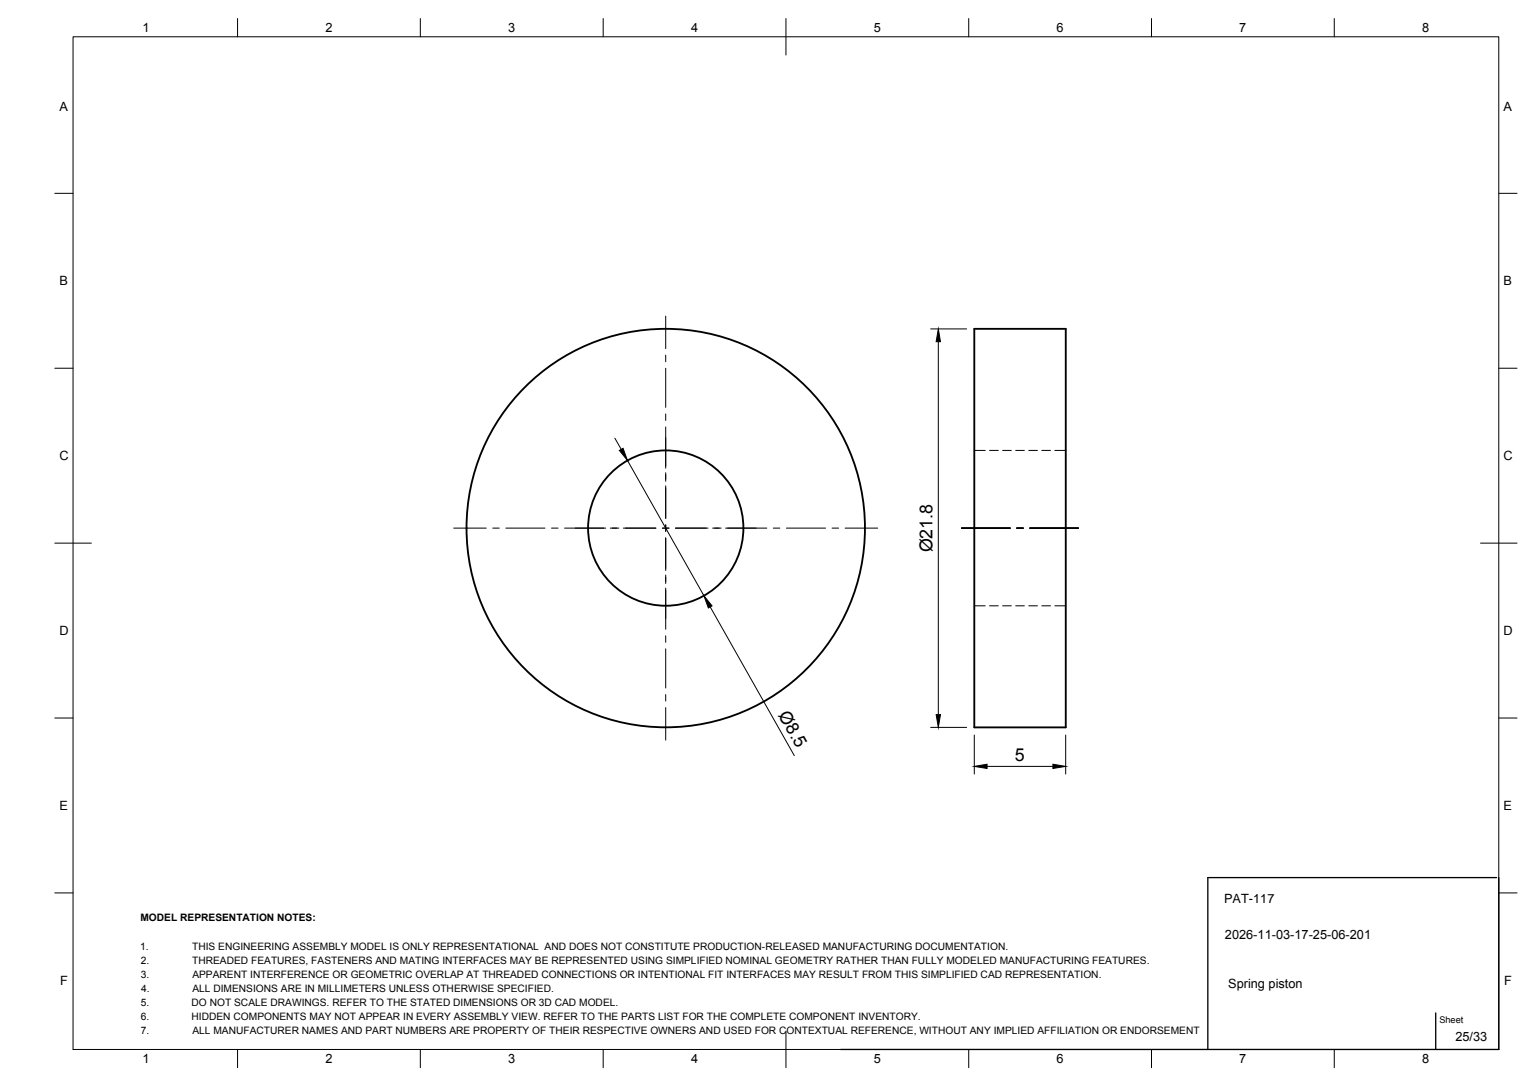
ISO-10303-21;
HEADER;
/* Generated by software containing ST-Developer
 * from STEP Tools, Inc. (www.steptools.com) 
 */

FILE_DESCRIPTION(
/* description */ ('Counterbalanced vertical column'),
/* implementation_level */ '2;1');

FILE_NAME(
/* name */ 'Spring piston.step',
/* time_stamp */ '2026-10-29T16:47:22-07:00',
/* author */ (''),
/* organization */ (''),
/* preprocessor_version */ 'ST-DEVELOPER v20.2',
/* originating_system */ 'Autodesk Translation Framework v15.17.0.0',
/* authorisation */ '');

FILE_SCHEMA (('AUTOMOTIVE_DESIGN { 1 0 10303 214 3 1 1 }'));
ENDSEC;

DATA;
#10=MECHANICAL_DESIGN_GEOMETRIC_PRESENTATION_REPRESENTATION('',(#374),#15040);
#304=SHAPE_REPRESENTATION_RELATIONSHIP('SRR','None',#15209,#339);
#339=ADVANCED_BREP_SHAPE_REPRESENTATION('',(#407),#15028);
#374=STYLED_ITEM('',(#15457),#407);
#407=MANIFOLD_SOLID_BREP('Body1',#7099);
#514=FACE_BOUND('',#1625,.T.);
#515=FACE_BOUND('',#1627,.T.);
#741=PLANE('',#7990);
#742=PLANE('',#7991);
#1119=FACE_OUTER_BOUND('',#1622,.T.);
#1120=FACE_OUTER_BOUND('',#1623,.T.);
#1121=FACE_OUTER_BOUND('',#1624,.T.);
#1122=FACE_OUTER_BOUND('',#1626,.T.);
#1622=EDGE_LOOP('',(#6090,#6091,#6092,#6093));
#1623=EDGE_LOOP('',(#6094,#6095,#6096,#6097));
#1624=EDGE_LOOP('',(#6098));
#1625=EDGE_LOOP('',(#6099));
#1626=EDGE_LOOP('',(#6100));
#1627=EDGE_LOOP('',(#6101));
#2235=LINE('',#14382,#2906);
#2236=LINE('',#14388,#2907);
#2906=VECTOR('',#9681,0.425);
#2907=VECTOR('',#9688,1.09);
#3251=CIRCLE('',#7985,0.425);
#3252=CIRCLE('',#7986,0.425);
#3253=CIRCLE('',#7988,1.09);
#3254=CIRCLE('',#7989,1.09);
#3736=VERTEX_POINT('',#14379);
#3737=VERTEX_POINT('',#14381);
#3738=VERTEX_POINT('',#14385);
#3739=VERTEX_POINT('',#14387);
#4546=EDGE_CURVE('',#3736,#3736,#3251,.T.);
#4547=EDGE_CURVE('',#3736,#3737,#2235,.T.);
#4548=EDGE_CURVE('',#3737,#3737,#3252,.T.);
#4549=EDGE_CURVE('',#3738,#3738,#3253,.T.);
#4550=EDGE_CURVE('',#3738,#3739,#2236,.T.);
#4551=EDGE_CURVE('',#3739,#3739,#3254,.T.);
#6090=ORIENTED_EDGE('',*,*,#4546,.F.);
#6091=ORIENTED_EDGE('',*,*,#4547,.T.);
#6092=ORIENTED_EDGE('',*,*,#4548,.F.);
#6093=ORIENTED_EDGE('',*,*,#4547,.F.);
#6094=ORIENTED_EDGE('',*,*,#4549,.F.);
#6095=ORIENTED_EDGE('',*,*,#4550,.T.);
#6096=ORIENTED_EDGE('',*,*,#4551,.T.);
#6097=ORIENTED_EDGE('',*,*,#4550,.F.);
#6098=ORIENTED_EDGE('',*,*,#4549,.T.);
#6099=ORIENTED_EDGE('',*,*,#4548,.T.);
#6100=ORIENTED_EDGE('',*,*,#4551,.F.);
#6101=ORIENTED_EDGE('',*,*,#4546,.T.);
#6648=CYLINDRICAL_SURFACE('',#7984,0.425);
#6649=CYLINDRICAL_SURFACE('',#7987,1.09);
#6961=ADVANCED_FACE('',(#1119),#6648,.F.);
#6962=ADVANCED_FACE('',(#1120),#6649,.T.);
#6963=ADVANCED_FACE('',(#1121,#514),#741,.T.);
#6964=ADVANCED_FACE('',(#1122,#515),#742,.F.);
#7099=CLOSED_SHELL('',(#6961,#6962,#6963,#6964));
#7983=AXIS2_PLACEMENT_3D('',#14377,#9675,#9676);
#7984=AXIS2_PLACEMENT_3D('',#14378,#9677,#9678);
#7985=AXIS2_PLACEMENT_3D('',#14380,#9679,#9680);
#7986=AXIS2_PLACEMENT_3D('',#14383,#9682,#9683);
#7987=AXIS2_PLACEMENT_3D('',#14384,#9684,#9685);
#7988=AXIS2_PLACEMENT_3D('',#14386,#9686,#9687);
#7989=AXIS2_PLACEMENT_3D('',#14389,#9689,#9690);
#7990=AXIS2_PLACEMENT_3D('',#14390,#9691,#9692);
#7991=AXIS2_PLACEMENT_3D('',#14391,#9693,#9694);
#9675=DIRECTION('axis',(0.,0.,1.));
#9676=DIRECTION('refdir',(1.,0.,0.));
#9677=DIRECTION('center_axis',(0.,0.,1.));
#9678=DIRECTION('ref_axis',(1.,0.,0.));
#9679=DIRECTION('center_axis',(0.,0.,1.));
#9680=DIRECTION('ref_axis',(1.,0.,0.));
#9681=DIRECTION('',(0.,0.,1.));
#9682=DIRECTION('center_axis',(0.,0.,-1.));
#9683=DIRECTION('ref_axis',(1.,0.,0.));
#9684=DIRECTION('center_axis',(0.,0.,1.));
#9685=DIRECTION('ref_axis',(1.,0.,0.));
#9686=DIRECTION('center_axis',(0.,0.,1.));
#9687=DIRECTION('ref_axis',(1.,0.,0.));
#9688=DIRECTION('',(0.,0.,-1.));
#9689=DIRECTION('center_axis',(0.,0.,1.));
#9690=DIRECTION('ref_axis',(1.,0.,0.));
#9691=DIRECTION('center_axis',(0.,0.,1.));
#9692=DIRECTION('ref_axis',(1.,0.,0.));
#9693=DIRECTION('center_axis',(0.,0.,1.));
#9694=DIRECTION('ref_axis',(1.,0.,0.));
#14377=CARTESIAN_POINT('',(0.,0.,0.));
#14378=CARTESIAN_POINT('Origin',(-7.,0.,4.9));
#14379=CARTESIAN_POINT('',(-7.425,-5.20474889637625E-17,5.));
#14380=CARTESIAN_POINT('Origin',(-7.,0.,5.));
#14381=CARTESIAN_POINT('',(-7.425,5.20474889637625E-17,5.5));
#14382=CARTESIAN_POINT('',(-7.425,-5.20474889637625E-17,4.9));
#14383=CARTESIAN_POINT('Origin',(-7.,0.,5.5));
#14384=CARTESIAN_POINT('Origin',(-7.,0.,5.));
#14385=CARTESIAN_POINT('',(-8.09,-1.33486501107061E-16,5.5));
#14386=CARTESIAN_POINT('Origin',(-7.,0.,5.5));
#14387=CARTESIAN_POINT('',(-8.09,-1.33486501107061E-16,5.));
#14388=CARTESIAN_POINT('',(-8.09,-1.33486501107061E-16,5.));
#14389=CARTESIAN_POINT('Origin',(-7.,0.,5.));
#14390=CARTESIAN_POINT('Origin',(-7.,0.,5.5));
#14391=CARTESIAN_POINT('Origin',(-7.,0.,5.));
#14988=UNCERTAINTY_MEASURE_WITH_UNIT(LENGTH_MEASURE(0.001),#15041,
'DISTANCE_ACCURACY_VALUE',
'Maximum model space distance between geometric entities at asserted c
onnectivities');
#15000=UNCERTAINTY_MEASURE_WITH_UNIT(LENGTH_MEASURE(0.001),#15041,
'DISTANCE_ACCURACY_VALUE',
'Maximum model space distance between geometric entities at asserted c
onnectivities');
#15028=(
GEOMETRIC_REPRESENTATION_CONTEXT(3)
GLOBAL_UNCERTAINTY_ASSIGNED_CONTEXT((#14988))
GLOBAL_UNIT_ASSIGNED_CONTEXT((#15041,#15043,#15044))
REPRESENTATION_CONTEXT('','3D')
);
#15040=(
GEOMETRIC_REPRESENTATION_CONTEXT(3)
GLOBAL_UNCERTAINTY_ASSIGNED_CONTEXT((#15000))
GLOBAL_UNIT_ASSIGNED_CONTEXT((#15041,#15043,#15044))
REPRESENTATION_CONTEXT('','3D')
);
#15041=(
LENGTH_UNIT()
NAMED_UNIT(*)
SI_UNIT(.CENTI.,.METRE.)
);
#15043=(
NAMED_UNIT(*)
PLANE_ANGLE_UNIT()
SI_UNIT($,.RADIAN.)
);
#15044=(
NAMED_UNIT(*)
SI_UNIT($,.STERADIAN.)
SOLID_ANGLE_UNIT()
);
#15072=SHAPE_DEFINITION_REPRESENTATION(#15111,#15209);
#15111=PRODUCT_DEFINITION_SHAPE('',$,#15249);
#15209=SHAPE_REPRESENTATION('',(#7983),#15028);
#15221=PRODUCT_DEFINITION_CONTEXT('part definition',#15340,'design');
#15249=PRODUCT_DEFINITION('Spring piston','Spring piston',#15288,#15221);
#15288=PRODUCT_DEFINITION_FORMATION('',$,#15369);
#15340=APPLICATION_CONTEXT(
'Core Data for Automotive Mechanical Design Process');
#15341=PRODUCT_CONTEXT('part definition',#15340,'mechanical');
#15369=PRODUCT('Spring piston','Spring piston','Spring piston',(#15341));
#15451=COLOUR_RGB('Grey',0.48,0.52,0.57);
#15452=FILL_AREA_STYLE_COLOUR('',#15451);
#15453=FILL_AREA_STYLE('',(#15452));
#15454=SURFACE_STYLE_FILL_AREA(#15453);
#15455=SURFACE_SIDE_STYLE('',(#15454));
#15456=SURFACE_STYLE_USAGE(.BOTH.,#15455);
#15457=PRESENTATION_STYLE_ASSIGNMENT((#15456));
ENDSEC;
END-ISO-10303-21;
